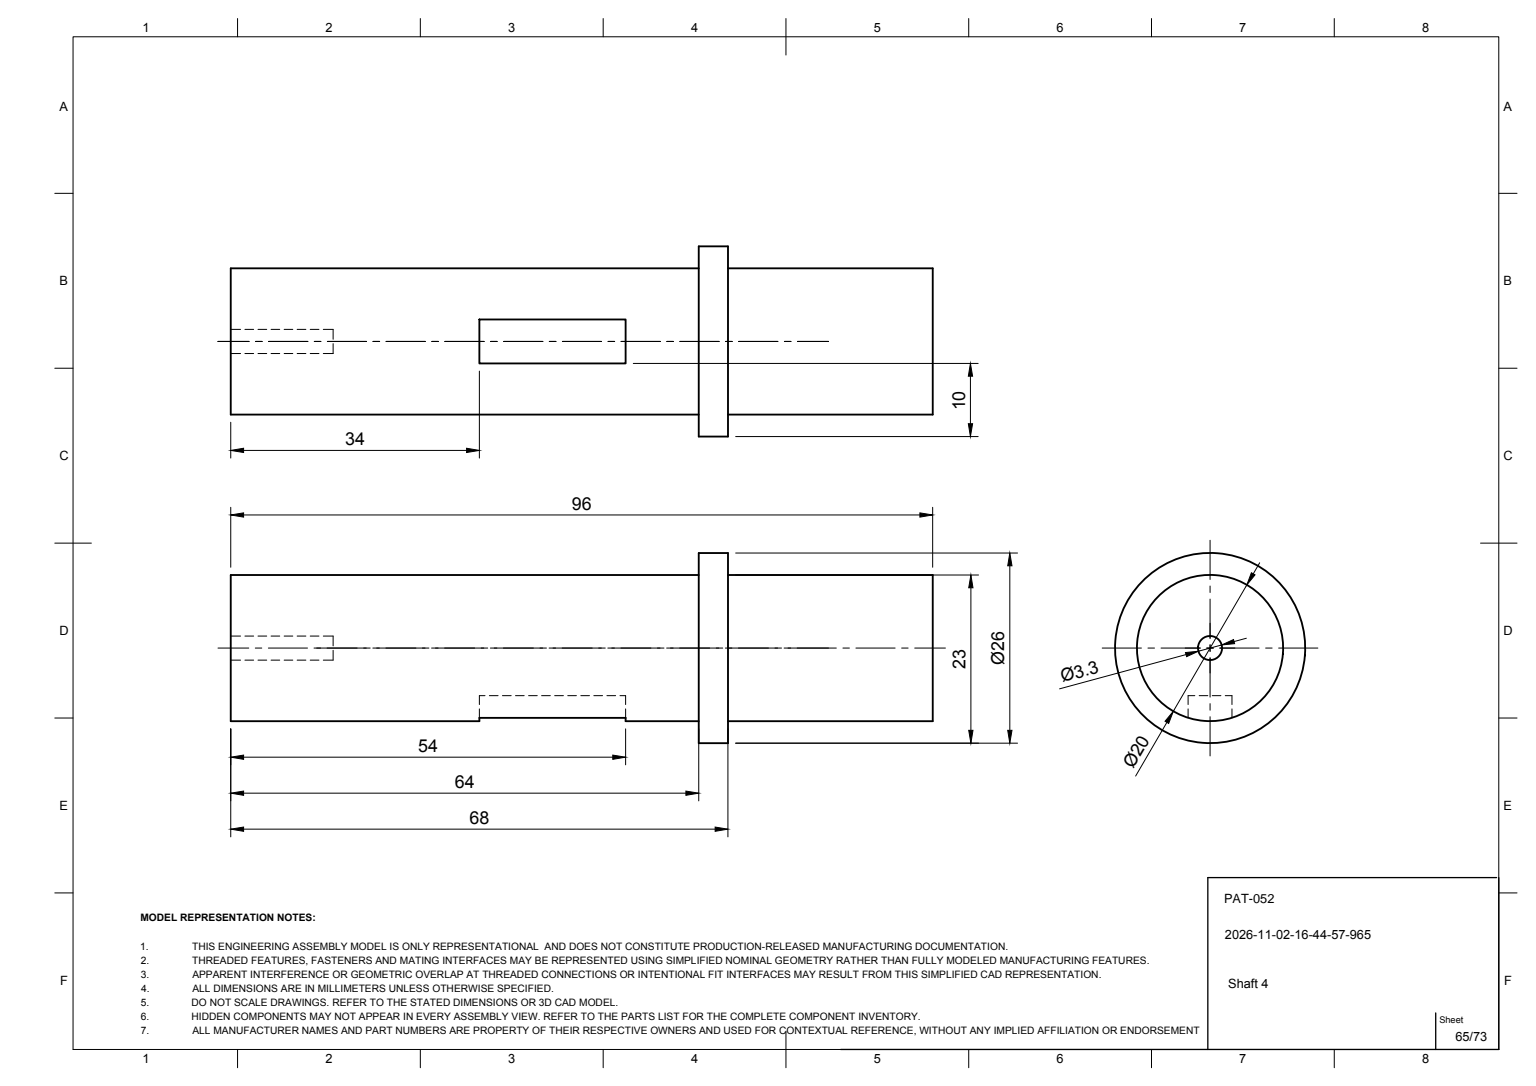
ISO-10303-21;
HEADER;
/* Generated by software containing ST-Developer
 * from STEP Tools, Inc. (www.steptools.com) 
 */

FILE_DESCRIPTION(
/* description */ ('Hand-crank gear train demonstrator'),
/* implementation_level */ '2;1');

FILE_NAME(
/* name */ 'Shaft 4.step',
/* time_stamp */ '2026-10-28T03:22:13-07:00',
/* author */ (''),
/* organization */ (''),
/* preprocessor_version */ 'ST-DEVELOPER v20.2',
/* originating_system */ 'Autodesk Translation Framework v15.17.0.0',
/* authorisation */ '');

FILE_SCHEMA (('AUTOMOTIVE_DESIGN { 1 0 10303 214 3 1 1 }'));
ENDSEC;

DATA;
#10=MECHANICAL_DESIGN_GEOMETRIC_PRESENTATION_REPRESENTATION('',(#1255),#62758);
#1112=SHAPE_REPRESENTATION_RELATIONSHIP('SRR','None',#63090,#1176);
#1176=ADVANCED_BREP_SHAPE_REPRESENTATION('',(#1330),#62744);
#1255=STYLED_ITEM('',(#63462),#1330);
#1330=MANIFOLD_SOLID_BREP('Body1',#16439);
#1603=FACE_BOUND('',#4001,.T.);
#1604=FACE_BOUND('',#4003,.T.);
#1605=FACE_BOUND('',#4007,.T.);
#1606=FACE_BOUND('',#4009,.T.);
#2013=PLANE('',#18380);
#2014=PLANE('',#18381);
#2015=PLANE('',#18382);
#2016=PLANE('',#18384);
#2017=PLANE('',#18385);
#2018=PLANE('',#18386);
#2019=PLANE('',#18388);
#2020=PLANE('',#18391);
#2021=PLANE('',#18399);
#2022=PLANE('',#18400);
#2796=FACE_OUTER_BOUND('',#3993,.T.);
#2797=FACE_OUTER_BOUND('',#3994,.T.);
#2798=FACE_OUTER_BOUND('',#3995,.T.);
#2799=FACE_OUTER_BOUND('',#3996,.T.);
#2800=FACE_OUTER_BOUND('',#3997,.T.);
#2801=FACE_OUTER_BOUND('',#3998,.T.);
#2802=FACE_OUTER_BOUND('',#3999,.T.);
#2803=FACE_OUTER_BOUND('',#4000,.T.);
#2804=FACE_OUTER_BOUND('',#4002,.T.);
#2805=FACE_OUTER_BOUND('',#4004,.T.);
#2806=FACE_OUTER_BOUND('',#4005,.T.);
#2807=FACE_OUTER_BOUND('',#4006,.T.);
#2808=FACE_OUTER_BOUND('',#4008,.T.);
#2809=FACE_OUTER_BOUND('',#4010,.T.);
#3993=EDGE_LOOP('',(#13813,#13814,#13815,#13816));
#3994=EDGE_LOOP('',(#13817));
#3995=EDGE_LOOP('',(#13818,#13819,#13820,#13821));
#3996=EDGE_LOOP('',(#13822,#13823,#13824,#13825));
#3997=EDGE_LOOP('',(#13826,#13827,#13828,#13829));
#3998=EDGE_LOOP('',(#13830,#13831,#13832,#13833));
#3999=EDGE_LOOP('',(#13834,#13835,#13836,#13837));
#4000=EDGE_LOOP('',(#13838));
#4001=EDGE_LOOP('',(#13839));
#4002=EDGE_LOOP('',(#13840));
#4003=EDGE_LOOP('',(#13841));
#4004=EDGE_LOOP('',(#13842,#13843,#13844,#13845));
#4005=EDGE_LOOP('',(#13846,#13847,#13848,#13849));
#4006=EDGE_LOOP('',(#13850,#13851,#13852,#13853));
#4007=EDGE_LOOP('',(#13854,#13855,#13856,#13857));
#4008=EDGE_LOOP('',(#13858));
#4009=EDGE_LOOP('',(#13859));
#4010=EDGE_LOOP('',(#13860));
#5135=LINE('',#38428,#6267);
#5136=LINE('',#38434,#6268);
#5137=LINE('',#38436,#6269);
#5138=LINE('',#38438,#6270);
#5139=LINE('',#38439,#6271);
#5140=LINE('',#38444,#6272);
#5141=LINE('',#38445,#6273);
#5142=LINE('',#38448,#6274);
#5143=LINE('',#38450,#6275);
#5144=LINE('',#38451,#6276);
#5145=LINE('',#38453,#6277);
#5146=LINE('',#38467,#6278);
#5147=LINE('',#38470,#6279);
#5148=LINE('',#38475,#6280);
#6267=VECTOR('',#22122,0.164999999999999);
#6268=VECTOR('',#22129,1.);
#6269=VECTOR('',#22130,1.);
#6270=VECTOR('',#22131,1.);
#6271=VECTOR('',#22132,1.);
#6272=VECTOR('',#22137,1.);
#6273=VECTOR('',#22138,1.);
#6274=VECTOR('',#22141,1.);
#6275=VECTOR('',#22142,1.);
#6276=VECTOR('',#22143,1.);
#6277=VECTOR('',#22146,1.);
#6278=VECTOR('',#22165,1.3);
#6279=VECTOR('',#22168,1.);
#6280=VECTOR('',#22175,1.);
#7066=CIRCLE('',#18378,0.164999999999999);
#7067=CIRCLE('',#18379,0.164999999999999);
#7068=CIRCLE('',#18383,1.);
#7069=CIRCLE('',#18387,1.);
#7070=CIRCLE('',#18389,1.3);
#7071=CIRCLE('',#18390,1.);
#7072=CIRCLE('',#18392,1.3);
#7073=CIRCLE('',#18393,1.);
#7074=CIRCLE('',#18396,1.);
#7075=CIRCLE('',#18398,1.);
#8219=VERTEX_POINT('',#38425);
#8220=VERTEX_POINT('',#38427);
#8221=VERTEX_POINT('',#38432);
#8222=VERTEX_POINT('',#38433);
#8223=VERTEX_POINT('',#38435);
#8224=VERTEX_POINT('',#38437);
#8225=VERTEX_POINT('',#38441);
#8226=VERTEX_POINT('',#38443);
#8227=VERTEX_POINT('',#38447);
#8228=VERTEX_POINT('',#38449);
#8229=VERTEX_POINT('',#38457);
#8230=VERTEX_POINT('',#38459);
#8231=VERTEX_POINT('',#38462);
#8232=VERTEX_POINT('',#38464);
#8233=VERTEX_POINT('',#38469);
#8234=VERTEX_POINT('',#38473);
#10158=EDGE_CURVE('',#8219,#8219,#7066,.T.);
#10159=EDGE_CURVE('',#8219,#8220,#5135,.T.);
#10160=EDGE_CURVE('',#8220,#8220,#7067,.T.);
#10161=EDGE_CURVE('',#8221,#8222,#5136,.T.);
#10162=EDGE_CURVE('',#8221,#8223,#5137,.T.);
#10163=EDGE_CURVE('',#8224,#8223,#5138,.T.);
#10164=EDGE_CURVE('',#8224,#8222,#5139,.T.);
#10165=EDGE_CURVE('',#8222,#8225,#7068,.T.);
#10166=EDGE_CURVE('',#8226,#8224,#5140,.T.);
#10167=EDGE_CURVE('',#8225,#8226,#5141,.T.);
#10168=EDGE_CURVE('',#8225,#8227,#5142,.T.);
#10169=EDGE_CURVE('',#8226,#8228,#5143,.T.);
#10170=EDGE_CURVE('',#8228,#8227,#5144,.T.);
#10171=EDGE_CURVE('',#8223,#8228,#5145,.T.);
#10172=EDGE_CURVE('',#8227,#8221,#7069,.T.);
#10173=EDGE_CURVE('',#8229,#8229,#7070,.T.);
#10174=EDGE_CURVE('',#8230,#8230,#7071,.T.);
#10175=EDGE_CURVE('',#8231,#8231,#7072,.T.);
#10176=EDGE_CURVE('',#8232,#8232,#7073,.T.);
#10177=EDGE_CURVE('',#8229,#8231,#5146,.T.);
#10178=EDGE_CURVE('',#8232,#8233,#5147,.T.);
#10179=EDGE_CURVE('',#8233,#8233,#7074,.T.);
#10180=EDGE_CURVE('',#8234,#8234,#7075,.T.);
#10181=EDGE_CURVE('',#8234,#8230,#5148,.T.);
#13813=ORIENTED_EDGE('',*,*,#10158,.F.);
#13814=ORIENTED_EDGE('',*,*,#10159,.T.);
#13815=ORIENTED_EDGE('',*,*,#10160,.F.);
#13816=ORIENTED_EDGE('',*,*,#10159,.F.);
#13817=ORIENTED_EDGE('',*,*,#10158,.T.);
#13818=ORIENTED_EDGE('',*,*,#10161,.F.);
#13819=ORIENTED_EDGE('',*,*,#10162,.T.);
#13820=ORIENTED_EDGE('',*,*,#10163,.F.);
#13821=ORIENTED_EDGE('',*,*,#10164,.T.);
#13822=ORIENTED_EDGE('',*,*,#10165,.F.);
#13823=ORIENTED_EDGE('',*,*,#10164,.F.);
#13824=ORIENTED_EDGE('',*,*,#10166,.F.);
#13825=ORIENTED_EDGE('',*,*,#10167,.F.);
#13826=ORIENTED_EDGE('',*,*,#10168,.F.);
#13827=ORIENTED_EDGE('',*,*,#10167,.T.);
#13828=ORIENTED_EDGE('',*,*,#10169,.T.);
#13829=ORIENTED_EDGE('',*,*,#10170,.T.);
#13830=ORIENTED_EDGE('',*,*,#10166,.T.);
#13831=ORIENTED_EDGE('',*,*,#10163,.T.);
#13832=ORIENTED_EDGE('',*,*,#10171,.T.);
#13833=ORIENTED_EDGE('',*,*,#10169,.F.);
#13834=ORIENTED_EDGE('',*,*,#10172,.F.);
#13835=ORIENTED_EDGE('',*,*,#10170,.F.);
#13836=ORIENTED_EDGE('',*,*,#10171,.F.);
#13837=ORIENTED_EDGE('',*,*,#10162,.F.);
#13838=ORIENTED_EDGE('',*,*,#10173,.T.);
#13839=ORIENTED_EDGE('',*,*,#10174,.F.);
#13840=ORIENTED_EDGE('',*,*,#10175,.F.);
#13841=ORIENTED_EDGE('',*,*,#10176,.F.);
#13842=ORIENTED_EDGE('',*,*,#10173,.F.);
#13843=ORIENTED_EDGE('',*,*,#10177,.T.);
#13844=ORIENTED_EDGE('',*,*,#10175,.T.);
#13845=ORIENTED_EDGE('',*,*,#10177,.F.);
#13846=ORIENTED_EDGE('',*,*,#10176,.T.);
#13847=ORIENTED_EDGE('',*,*,#10178,.T.);
#13848=ORIENTED_EDGE('',*,*,#10179,.T.);
#13849=ORIENTED_EDGE('',*,*,#10178,.F.);
#13850=ORIENTED_EDGE('',*,*,#10180,.F.);
#13851=ORIENTED_EDGE('',*,*,#10181,.T.);
#13852=ORIENTED_EDGE('',*,*,#10174,.T.);
#13853=ORIENTED_EDGE('',*,*,#10181,.F.);
#13854=ORIENTED_EDGE('',*,*,#10168,.T.);
#13855=ORIENTED_EDGE('',*,*,#10172,.T.);
#13856=ORIENTED_EDGE('',*,*,#10161,.T.);
#13857=ORIENTED_EDGE('',*,*,#10165,.T.);
#13858=ORIENTED_EDGE('',*,*,#10180,.T.);
#13859=ORIENTED_EDGE('',*,*,#10160,.T.);
#13860=ORIENTED_EDGE('',*,*,#10179,.F.);
#15366=CYLINDRICAL_SURFACE('',#18377,0.164999999999999);
#15367=CYLINDRICAL_SURFACE('',#18394,1.3);
#15368=CYLINDRICAL_SURFACE('',#18395,1.);
#15369=CYLINDRICAL_SURFACE('',#18397,1.);
#16106=ADVANCED_FACE('',(#2796),#15366,.F.);
#16107=ADVANCED_FACE('',(#2797),#2013,.T.);
#16108=ADVANCED_FACE('',(#2798),#2014,.F.);
#16109=ADVANCED_FACE('',(#2799),#2015,.T.);
#16110=ADVANCED_FACE('',(#2800),#2016,.F.);
#16111=ADVANCED_FACE('',(#2801),#2017,.F.);
#16112=ADVANCED_FACE('',(#2802),#2018,.F.);
#16113=ADVANCED_FACE('',(#2803,#1603),#2019,.T.);
#16114=ADVANCED_FACE('',(#2804,#1604),#2020,.F.);
#16115=ADVANCED_FACE('',(#2805),#15367,.T.);
#16116=ADVANCED_FACE('',(#2806),#15368,.T.);
#16117=ADVANCED_FACE('',(#2807,#1605),#15369,.T.);
#16118=ADVANCED_FACE('',(#2808,#1606),#2021,.T.);
#16119=ADVANCED_FACE('',(#2809),#2022,.F.);
#16439=CLOSED_SHELL('',(#16106,#16107,#16108,#16109,#16110,#16111,#16112,
#16113,#16114,#16115,#16116,#16117,#16118,#16119));
#18376=AXIS2_PLACEMENT_3D('',#38423,#22116,#22117);
#18377=AXIS2_PLACEMENT_3D('',#38424,#22118,#22119);
#18378=AXIS2_PLACEMENT_3D('',#38426,#22120,#22121);
#18379=AXIS2_PLACEMENT_3D('',#38429,#22123,#22124);
#18380=AXIS2_PLACEMENT_3D('',#38430,#22125,#22126);
#18381=AXIS2_PLACEMENT_3D('',#38431,#22127,#22128);
#18382=AXIS2_PLACEMENT_3D('',#38440,#22133,#22134);
#18383=AXIS2_PLACEMENT_3D('',#38442,#22135,#22136);
#18384=AXIS2_PLACEMENT_3D('',#38446,#22139,#22140);
#18385=AXIS2_PLACEMENT_3D('',#38452,#22144,#22145);
#18386=AXIS2_PLACEMENT_3D('',#38454,#22147,#22148);
#18387=AXIS2_PLACEMENT_3D('',#38455,#22149,#22150);
#18388=AXIS2_PLACEMENT_3D('',#38456,#22151,#22152);
#18389=AXIS2_PLACEMENT_3D('',#38458,#22153,#22154);
#18390=AXIS2_PLACEMENT_3D('',#38460,#22155,#22156);
#18391=AXIS2_PLACEMENT_3D('',#38461,#22157,#22158);
#18392=AXIS2_PLACEMENT_3D('',#38463,#22159,#22160);
#18393=AXIS2_PLACEMENT_3D('',#38465,#22161,#22162);
#18394=AXIS2_PLACEMENT_3D('',#38466,#22163,#22164);
#18395=AXIS2_PLACEMENT_3D('',#38468,#22166,#22167);
#18396=AXIS2_PLACEMENT_3D('',#38471,#22169,#22170);
#18397=AXIS2_PLACEMENT_3D('',#38472,#22171,#22172);
#18398=AXIS2_PLACEMENT_3D('',#38474,#22173,#22174);
#18399=AXIS2_PLACEMENT_3D('',#38476,#22176,#22177);
#18400=AXIS2_PLACEMENT_3D('',#38477,#22178,#22179);
#22116=DIRECTION('axis',(0.,0.,1.));
#22117=DIRECTION('refdir',(1.,0.,0.));
#22118=DIRECTION('center_axis',(0.,1.,0.));
#22119=DIRECTION('ref_axis',(1.,0.,0.));
#22120=DIRECTION('center_axis',(0.,1.,0.));
#22121=DIRECTION('ref_axis',(1.,0.,0.));
#22122=DIRECTION('',(0.,1.,0.));
#22123=DIRECTION('center_axis',(0.,-1.,0.));
#22124=DIRECTION('ref_axis',(1.,0.,0.));
#22125=DIRECTION('center_axis',(0.,1.,0.));
#22126=DIRECTION('ref_axis',(1.,0.,0.));
#22127=DIRECTION('center_axis',(-1.,0.,0.));
#22128=DIRECTION('ref_axis',(0.,0.,1.));
#22129=DIRECTION('',(0.,-1.,0.));
#22130=DIRECTION('',(0.,0.,1.));
#22131=DIRECTION('',(0.,1.,0.));
#22132=DIRECTION('',(0.,0.,-1.));
#22133=DIRECTION('center_axis',(0.,1.,0.));
#22134=DIRECTION('ref_axis',(1.,0.,0.));
#22135=DIRECTION('center_axis',(0.,-1.,0.));
#22136=DIRECTION('ref_axis',(1.,0.,0.));
#22137=DIRECTION('',(-1.,0.,0.));
#22138=DIRECTION('',(0.,0.,1.));
#22139=DIRECTION('center_axis',(1.,0.,0.));
#22140=DIRECTION('ref_axis',(0.,0.,-1.));
#22141=DIRECTION('',(0.,1.,0.));
#22142=DIRECTION('',(0.,1.,0.));
#22143=DIRECTION('',(0.,0.,-1.));
#22144=DIRECTION('center_axis',(0.,0.,1.));
#22145=DIRECTION('ref_axis',(1.,0.,0.));
#22146=DIRECTION('',(1.,0.,0.));
#22147=DIRECTION('center_axis',(0.,1.,0.));
#22148=DIRECTION('ref_axis',(0.,0.,1.));
#22149=DIRECTION('center_axis',(0.,1.,0.));
#22150=DIRECTION('ref_axis',(1.,0.,0.));
#22151=DIRECTION('center_axis',(0.,1.,0.));
#22152=DIRECTION('ref_axis',(1.,0.,0.));
#22153=DIRECTION('center_axis',(0.,1.,0.));
#22154=DIRECTION('ref_axis',(1.,0.,0.));
#22155=DIRECTION('center_axis',(0.,1.,0.));
#22156=DIRECTION('ref_axis',(1.,0.,0.));
#22157=DIRECTION('center_axis',(0.,1.,0.));
#22158=DIRECTION('ref_axis',(1.,0.,0.));
#22159=DIRECTION('center_axis',(0.,1.,0.));
#22160=DIRECTION('ref_axis',(1.,0.,0.));
#22161=DIRECTION('center_axis',(0.,-1.,0.));
#22162=DIRECTION('ref_axis',(1.,0.,0.));
#22163=DIRECTION('center_axis',(0.,1.,0.));
#22164=DIRECTION('ref_axis',(1.,0.,0.));
#22165=DIRECTION('',(0.,-1.,0.));
#22166=DIRECTION('center_axis',(0.,1.,0.));
#22167=DIRECTION('ref_axis',(1.,0.,0.));
#22168=DIRECTION('',(0.,-1.,0.));
#22169=DIRECTION('center_axis',(0.,1.,0.));
#22170=DIRECTION('ref_axis',(1.,0.,0.));
#22171=DIRECTION('center_axis',(0.,1.,0.));
#22172=DIRECTION('ref_axis',(1.,0.,0.));
#22173=DIRECTION('center_axis',(0.,1.,0.));
#22174=DIRECTION('ref_axis',(1.,0.,0.));
#22175=DIRECTION('',(0.,-1.,0.));
#22176=DIRECTION('center_axis',(0.,1.,0.));
#22177=DIRECTION('ref_axis',(1.,0.,0.));
#22178=DIRECTION('center_axis',(0.,1.,0.));
#22179=DIRECTION('ref_axis',(1.,0.,0.));
#38423=CARTESIAN_POINT('',(0.,0.,0.));
#38424=CARTESIAN_POINT('Origin',(18.,4.6,9.));
#38425=CARTESIAN_POINT('',(17.835,4.6,9.));
#38426=CARTESIAN_POINT('Origin',(18.,4.6,9.));
#38427=CARTESIAN_POINT('',(17.835,6.,9.));
#38428=CARTESIAN_POINT('',(17.835,4.6,9.));
#38429=CARTESIAN_POINT('Origin',(18.,6.,9.));
#38430=CARTESIAN_POINT('Origin',(18.,4.6,9.));
#38431=CARTESIAN_POINT('Origin',(17.7,0.6,7.));
#38432=CARTESIAN_POINT('',(17.7,2.6,8.04606079858305));
#38433=CARTESIAN_POINT('',(17.7,0.6,8.04606079858305));
#38434=CARTESIAN_POINT('',(17.7,-3.6,8.04606079858305));
#38435=CARTESIAN_POINT('',(17.7,2.6,8.35));
#38436=CARTESIAN_POINT('',(17.7,2.6,8.35));
#38437=CARTESIAN_POINT('',(17.7,0.6,8.35));
#38438=CARTESIAN_POINT('',(17.7,0.6,8.35));
#38439=CARTESIAN_POINT('',(17.7,0.6,8.35));
#38440=CARTESIAN_POINT('Origin',(18.,0.6,7.675));
#38441=CARTESIAN_POINT('',(18.3,0.6,8.04606079858305));
#38442=CARTESIAN_POINT('Origin',(18.,0.6,9.));
#38443=CARTESIAN_POINT('',(18.3,0.6,8.35));
#38444=CARTESIAN_POINT('',(18.3,0.6,8.35));
#38445=CARTESIAN_POINT('',(18.3,0.6,7.));
#38446=CARTESIAN_POINT('Origin',(18.3,0.6,8.35));
#38447=CARTESIAN_POINT('',(18.3,2.6,8.04606079858305));
#38448=CARTESIAN_POINT('',(18.3,-3.6,8.04606079858305));
#38449=CARTESIAN_POINT('',(18.3,2.6,8.35));
#38450=CARTESIAN_POINT('',(18.3,0.6,8.35));
#38451=CARTESIAN_POINT('',(18.3,2.6,7.));
#38452=CARTESIAN_POINT('Origin',(17.7,0.6,8.35));
#38453=CARTESIAN_POINT('',(18.3,2.6,8.35));
#38454=CARTESIAN_POINT('Origin',(18.,2.6,7.675));
#38455=CARTESIAN_POINT('Origin',(18.,2.6,9.));
#38456=CARTESIAN_POINT('Origin',(18.,-0.4,9.));
#38457=CARTESIAN_POINT('',(16.7,-0.4,9.));
#38458=CARTESIAN_POINT('Origin',(18.,-0.4,9.));
#38459=CARTESIAN_POINT('',(17.,-0.4,9.));
#38460=CARTESIAN_POINT('Origin',(18.,-0.4,9.));
#38461=CARTESIAN_POINT('Origin',(18.,-0.8,9.));
#38462=CARTESIAN_POINT('',(16.7,-0.8,9.));
#38463=CARTESIAN_POINT('Origin',(18.,-0.8,9.));
#38464=CARTESIAN_POINT('',(17.,-0.8,9.));
#38465=CARTESIAN_POINT('Origin',(18.,-0.8,9.));
#38466=CARTESIAN_POINT('Origin',(18.,-0.8,9.));
#38467=CARTESIAN_POINT('',(16.7,-0.8,9.));
#38468=CARTESIAN_POINT('Origin',(18.,-3.6,9.));
#38469=CARTESIAN_POINT('',(17.,-3.6,9.));
#38470=CARTESIAN_POINT('',(17.,-3.6,9.));
#38471=CARTESIAN_POINT('Origin',(18.,-3.6,9.));
#38472=CARTESIAN_POINT('Origin',(18.,-3.6,9.));
#38473=CARTESIAN_POINT('',(17.,6.,9.));
#38474=CARTESIAN_POINT('Origin',(18.,6.,9.));
#38475=CARTESIAN_POINT('',(17.,-3.6,9.));
#38476=CARTESIAN_POINT('Origin',(18.,6.,9.));
#38477=CARTESIAN_POINT('Origin',(18.,-3.6,9.));
#62670=UNCERTAINTY_MEASURE_WITH_UNIT(LENGTH_MEASURE(0.001),#62759,
'DISTANCE_ACCURACY_VALUE',
'Maximum model space distance between geometric entities at asserted c
onnectivities');
#62684=UNCERTAINTY_MEASURE_WITH_UNIT(LENGTH_MEASURE(0.001),#62759,
'DISTANCE_ACCURACY_VALUE',
'Maximum model space distance between geometric entities at asserted c
onnectivities');
#62744=(
GEOMETRIC_REPRESENTATION_CONTEXT(3)
GLOBAL_UNCERTAINTY_ASSIGNED_CONTEXT((#62670))
GLOBAL_UNIT_ASSIGNED_CONTEXT((#62759,#62761,#62762))
REPRESENTATION_CONTEXT('','3D')
);
#62758=(
GEOMETRIC_REPRESENTATION_CONTEXT(3)
GLOBAL_UNCERTAINTY_ASSIGNED_CONTEXT((#62684))
GLOBAL_UNIT_ASSIGNED_CONTEXT((#62759,#62761,#62762))
REPRESENTATION_CONTEXT('','3D')
);
#62759=(
LENGTH_UNIT()
NAMED_UNIT(*)
SI_UNIT(.CENTI.,.METRE.)
);
#62761=(
NAMED_UNIT(*)
PLANE_ANGLE_UNIT()
SI_UNIT($,.RADIAN.)
);
#62762=(
NAMED_UNIT(*)
SI_UNIT($,.STERADIAN.)
SOLID_ANGLE_UNIT()
);
#62822=SHAPE_DEFINITION_REPRESENTATION(#62905,#63090);
#62905=PRODUCT_DEFINITION_SHAPE('',$,#63164);
#63090=SHAPE_REPRESENTATION('',(#18376),#62744);
#63104=PRODUCT_DEFINITION_CONTEXT('part definition',#63325,'design');
#63164=PRODUCT_DEFINITION('Shaft 4','Shaft 4',#63237,#63104);
#63237=PRODUCT_DEFINITION_FORMATION('',$,#63386);
#63325=APPLICATION_CONTEXT(
'Core Data for Automotive Mechanical Design Process');
#63326=PRODUCT_CONTEXT('part definition',#63325,'mechanical');
#63386=PRODUCT('Shaft 4','Shaft 4','Shaft 4',(#63326));
#63456=COLOUR_RGB('Grey',0.48,0.52,0.57);
#63457=FILL_AREA_STYLE_COLOUR('',#63456);
#63458=FILL_AREA_STYLE('',(#63457));
#63459=SURFACE_STYLE_FILL_AREA(#63458);
#63460=SURFACE_SIDE_STYLE('',(#63459));
#63461=SURFACE_STYLE_USAGE(.BOTH.,#63460);
#63462=PRESENTATION_STYLE_ASSIGNMENT((#63461));
ENDSEC;
END-ISO-10303-21;
